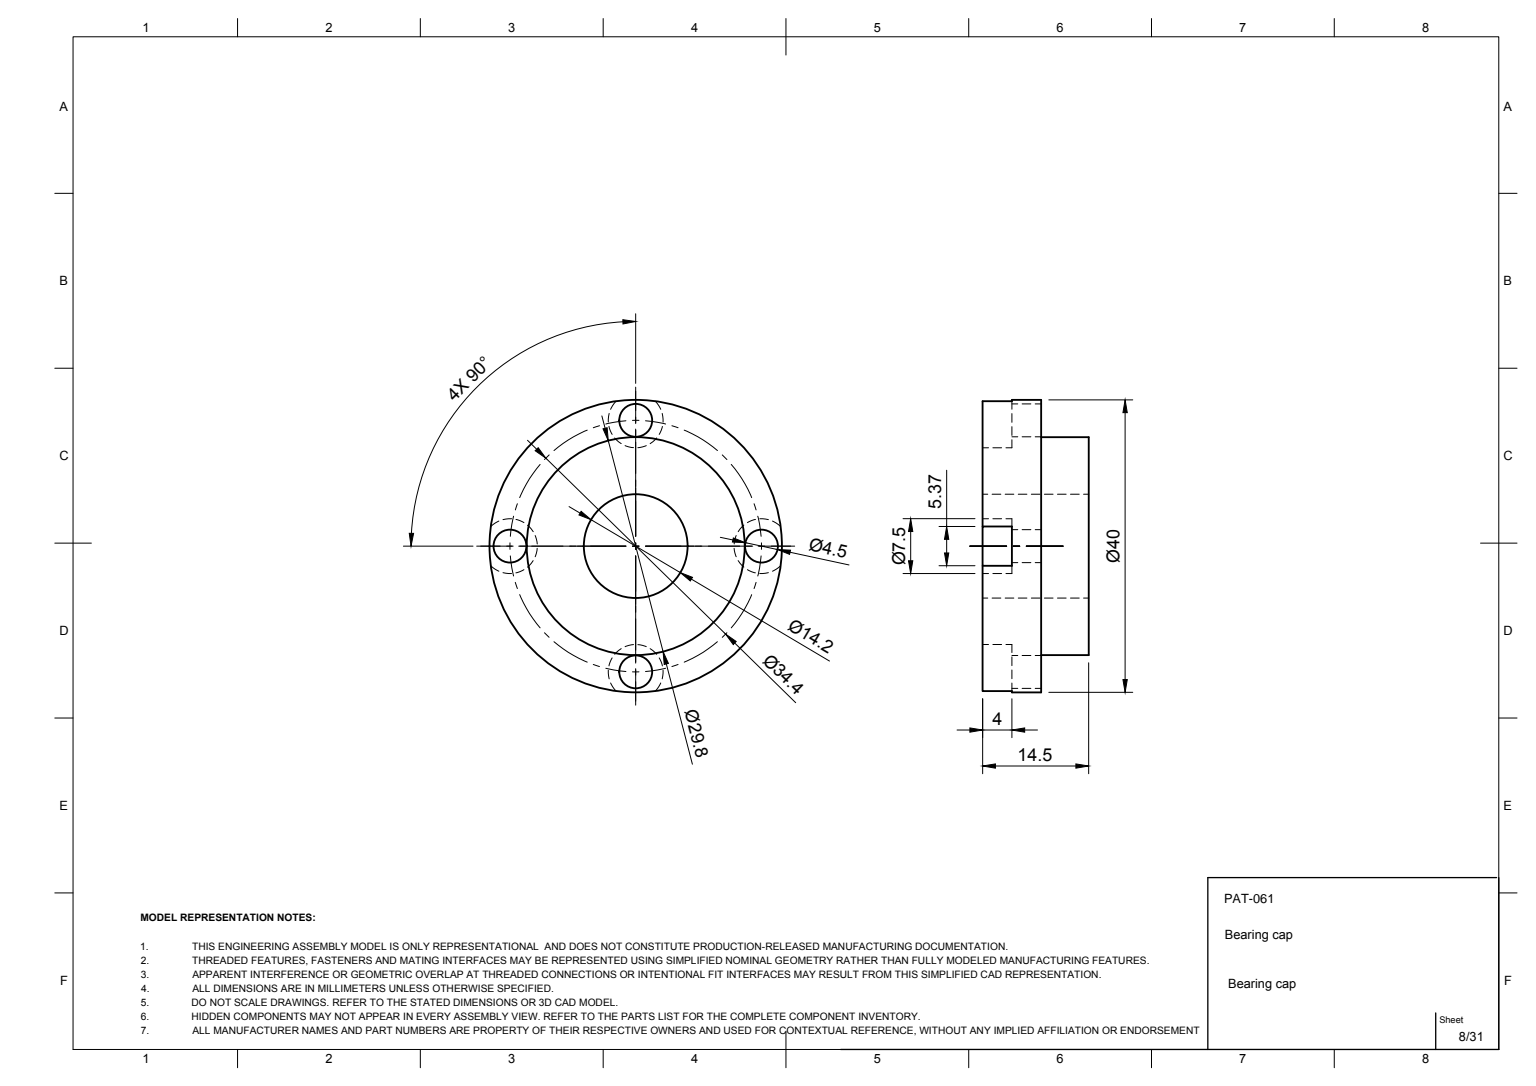
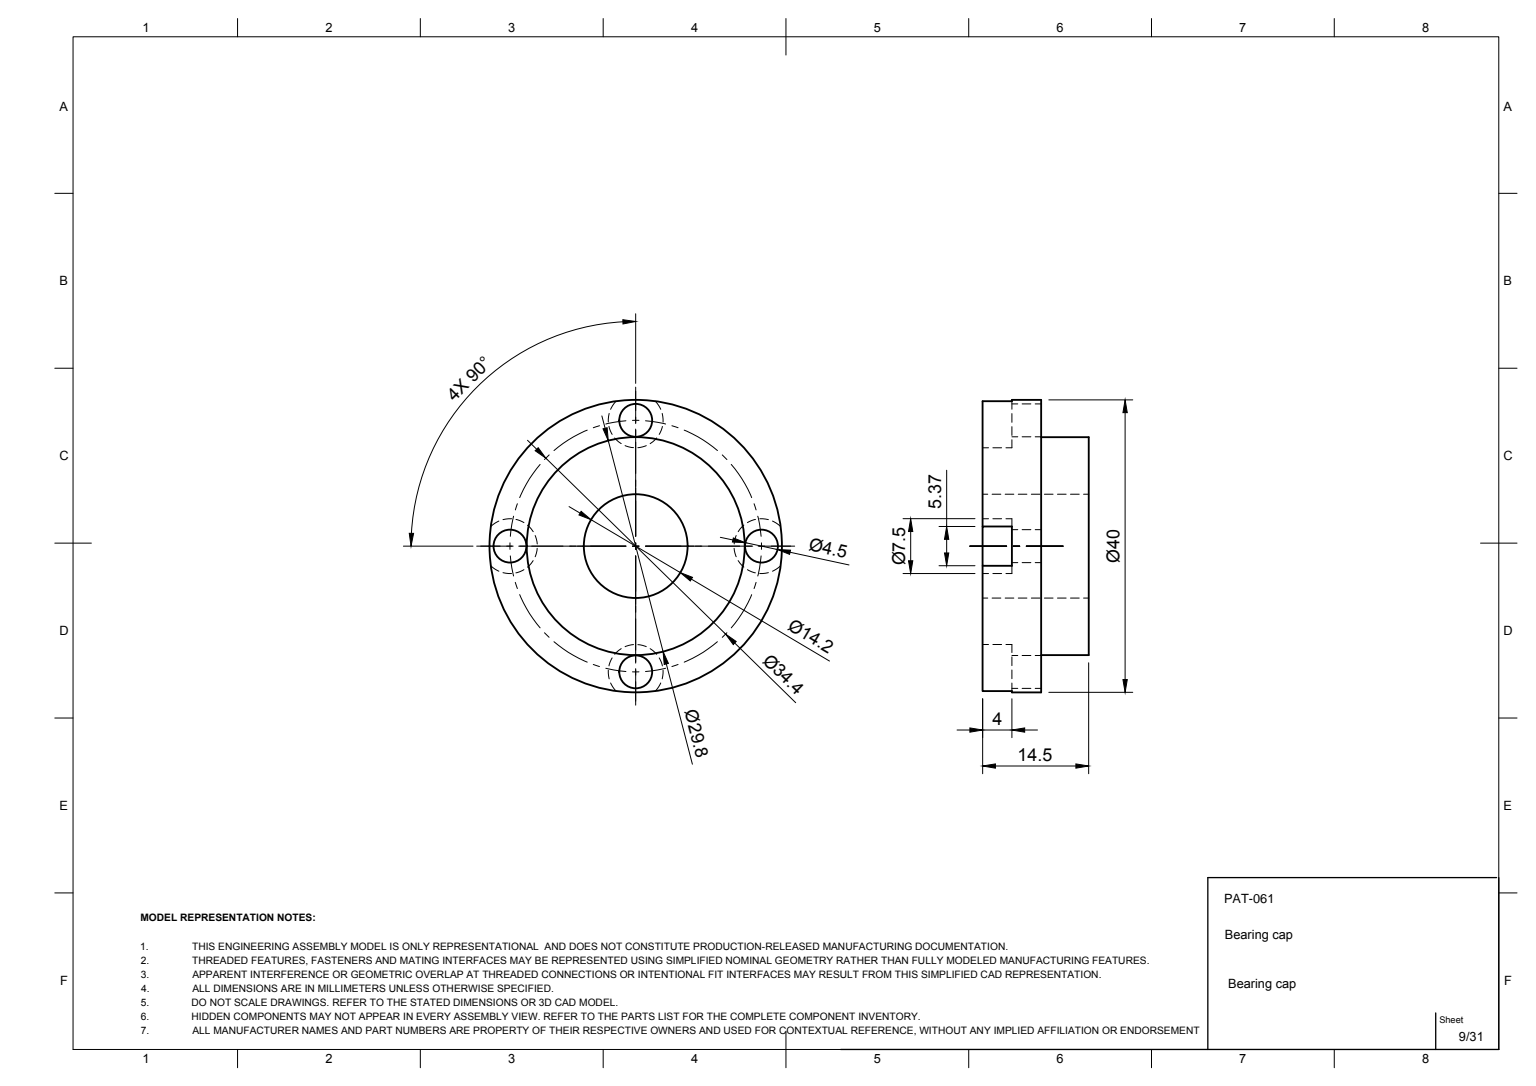
ISO-10303-21;
HEADER;
/* Generated by software containing ST-Developer
 * from STEP Tools, Inc. (www.steptools.com) 
 */

FILE_DESCRIPTION(
/* description */ ('Compact intermittent indexer'),
/* implementation_level */ '2;1');

FILE_NAME(
/* name */ 'Bearing cap.step',
/* time_stamp */ '2026-10-29T16:32:17-07:00',
/* author */ (''),
/* organization */ (''),
/* preprocessor_version */ 'ST-DEVELOPER v20.2',
/* originating_system */ 'Autodesk Translation Framework v15.17.0.0',
/* authorisation */ '');

FILE_SCHEMA (('AUTOMOTIVE_DESIGN { 1 0 10303 214 3 1 1 }'));
ENDSEC;

DATA;
#10=MECHANICAL_DESIGN_GEOMETRIC_PRESENTATION_REPRESENTATION('',(#260),#10837);
#212=SHAPE_REPRESENTATION_RELATIONSHIP('SRR','None',#10946,#236);
#236=ADVANCED_BREP_SHAPE_REPRESENTATION('',(#292),#10813);
#260=STYLED_ITEM('',(#11166),#292);
#292=MANIFOLD_SOLID_BREP('Body1',#5632);
#400=FACE_BOUND('',#1102,.T.);
#401=FACE_BOUND('',#1104,.T.);
#402=FACE_BOUND('',#1107,.T.);
#403=FACE_BOUND('',#1110,.T.);
#404=FACE_BOUND('',#1113,.T.);
#405=FACE_BOUND('',#1120,.T.);
#406=FACE_BOUND('',#1124,.T.);
#407=FACE_BOUND('',#1125,.T.);
#408=FACE_BOUND('',#1126,.T.);
#409=FACE_BOUND('',#1127,.T.);
#410=FACE_BOUND('',#1128,.T.);
#514=PLANE('',#6068);
#515=PLANE('',#6072);
#516=PLANE('',#6078);
#517=PLANE('',#6084);
#518=PLANE('',#6090);
#519=PLANE('',#6107);
#520=PLANE('',#6112);
#725=FACE_OUTER_BOUND('',#1100,.T.);
#726=FACE_OUTER_BOUND('',#1101,.T.);
#727=FACE_OUTER_BOUND('',#1103,.T.);
#728=FACE_OUTER_BOUND('',#1105,.T.);
#729=FACE_OUTER_BOUND('',#1106,.T.);
#730=FACE_OUTER_BOUND('',#1108,.T.);
#731=FACE_OUTER_BOUND('',#1109,.T.);
#732=FACE_OUTER_BOUND('',#1111,.T.);
#733=FACE_OUTER_BOUND('',#1112,.T.);
#734=FACE_OUTER_BOUND('',#1114,.T.);
#735=FACE_OUTER_BOUND('',#1115,.T.);
#736=FACE_OUTER_BOUND('',#1116,.T.);
#737=FACE_OUTER_BOUND('',#1117,.T.);
#738=FACE_OUTER_BOUND('',#1118,.T.);
#739=FACE_OUTER_BOUND('',#1119,.T.);
#740=FACE_OUTER_BOUND('',#1121,.T.);
#741=FACE_OUTER_BOUND('',#1122,.T.);
#742=FACE_OUTER_BOUND('',#1123,.T.);
#1100=EDGE_LOOP('',(#3984,#3985,#3986,#3987));
#1101=EDGE_LOOP('',(#3988,#3989,#3990));
#1102=EDGE_LOOP('',(#3991));
#1103=EDGE_LOOP('',(#3992,#3993));
#1104=EDGE_LOOP('',(#3994));
#1105=EDGE_LOOP('',(#3995,#3996,#3997,#3998));
#1106=EDGE_LOOP('',(#3999,#4000));
#1107=EDGE_LOOP('',(#4001));
#1108=EDGE_LOOP('',(#4002,#4003,#4004,#4005));
#1109=EDGE_LOOP('',(#4006,#4007));
#1110=EDGE_LOOP('',(#4008));
#1111=EDGE_LOOP('',(#4009,#4010,#4011,#4012));
#1112=EDGE_LOOP('',(#4013,#4014,#4015,#4016,#4017,#4018,#4019,#4020));
#1113=EDGE_LOOP('',(#4021));
#1114=EDGE_LOOP('',(#4022,#4023,#4024,#4025));
#1115=EDGE_LOOP('',(#4026,#4027,#4028,#4029));
#1116=EDGE_LOOP('',(#4030,#4031,#4032,#4033));
#1117=EDGE_LOOP('',(#4034,#4035,#4036,#4037));
#1118=EDGE_LOOP('',(#4038,#4039,#4040,#4041));
#1119=EDGE_LOOP('',(#4042));
#1120=EDGE_LOOP('',(#4043));
#1121=EDGE_LOOP('',(#4044,#4045,#4046,#4047));
#1122=EDGE_LOOP('',(#4048,#4049,#4050,#4051,#4052,#4053,#4054,#4055,#4056,
#4057,#4058,#4059,#4060,#4061,#4062,#4063,#4064,#4065,#4066,#4067));
#1123=EDGE_LOOP('',(#4068));
#1124=EDGE_LOOP('',(#4069));
#1125=EDGE_LOOP('',(#4070));
#1126=EDGE_LOOP('',(#4071));
#1127=EDGE_LOOP('',(#4072));
#1128=EDGE_LOOP('',(#4073));
#1510=LINE('',#8878,#1868);
#1511=LINE('',#8882,#1869);
#1512=LINE('',#8899,#1870);
#1513=LINE('',#8902,#1871);
#1514=LINE('',#8912,#1872);
#1515=LINE('',#8915,#1873);
#1516=LINE('',#8925,#1874);
#1517=LINE('',#8928,#1875);
#1518=LINE('',#8939,#1876);
#1519=LINE('',#8943,#1877);
#1520=LINE('',#8947,#1878);
#1521=LINE('',#8951,#1879);
#1522=LINE('',#8956,#1880);
#1523=LINE('',#8962,#1881);
#1524=LINE('',#8965,#1882);
#1868=VECTOR('',#7020,1.);
#1869=VECTOR('',#7023,1.);
#1870=VECTOR('',#7044,1.);
#1871=VECTOR('',#7047,1.);
#1872=VECTOR('',#7058,1.);
#1873=VECTOR('',#7061,1.);
#1874=VECTOR('',#7072,1.);
#1875=VECTOR('',#7075,1.);
#1876=VECTOR('',#7092,0.225);
#1877=VECTOR('',#7097,0.225);
#1878=VECTOR('',#7102,0.225);
#1879=VECTOR('',#7107,0.225);
#1880=VECTOR('',#7112,1.49);
#1881=VECTOR('',#7121,0.71);
#1882=VECTOR('',#7124,2.);
#2206=CIRCLE('',#6066,0.375);
#2207=CIRCLE('',#6067,0.375);
#2208=CIRCLE('',#6069,2.);
#2209=CIRCLE('',#6070,2.);
#2210=CIRCLE('',#6071,0.225);
#2211=CIRCLE('',#6073,2.);
#2212=CIRCLE('',#6074,0.375);
#2213=CIRCLE('',#6075,0.225);
#2214=CIRCLE('',#6077,0.375);
#2215=CIRCLE('',#6079,2.);
#2216=CIRCLE('',#6080,0.375);
#2217=CIRCLE('',#6081,0.225);
#2218=CIRCLE('',#6083,0.375);
#2219=CIRCLE('',#6085,2.);
#2220=CIRCLE('',#6086,0.375);
#2221=CIRCLE('',#6087,0.225);
#2222=CIRCLE('',#6089,0.375);
#2223=CIRCLE('',#6091,2.);
#2224=CIRCLE('',#6092,2.);
#2225=CIRCLE('',#6093,2.);
#2226=CIRCLE('',#6094,2.);
#2227=CIRCLE('',#6095,0.71);
#2228=CIRCLE('',#6097,0.225);
#2229=CIRCLE('',#6099,0.225);
#2230=CIRCLE('',#6101,0.225);
#2231=CIRCLE('',#6103,0.225);
#2232=CIRCLE('',#6105,1.49);
#2233=CIRCLE('',#6106,1.49);
#2234=CIRCLE('',#6108,0.71);
#2235=CIRCLE('',#6111,2.);
#2574=VERTEX_POINT('',#8876);
#2575=VERTEX_POINT('',#8877);
#2576=VERTEX_POINT('',#8879);
#2577=VERTEX_POINT('',#8881);
#2578=VERTEX_POINT('',#8885);
#2579=VERTEX_POINT('',#8888);
#2580=VERTEX_POINT('',#8891);
#2581=VERTEX_POINT('',#8892);
#2582=VERTEX_POINT('',#8895);
#2583=VERTEX_POINT('',#8898);
#2584=VERTEX_POINT('',#8900);
#2585=VERTEX_POINT('',#8904);
#2586=VERTEX_POINT('',#8905);
#2587=VERTEX_POINT('',#8908);
#2588=VERTEX_POINT('',#8911);
#2589=VERTEX_POINT('',#8913);
#2590=VERTEX_POINT('',#8917);
#2591=VERTEX_POINT('',#8918);
#2592=VERTEX_POINT('',#8921);
#2593=VERTEX_POINT('',#8924);
#2594=VERTEX_POINT('',#8926);
#2595=VERTEX_POINT('',#8934);
#2596=VERTEX_POINT('',#8937);
#2597=VERTEX_POINT('',#8941);
#2598=VERTEX_POINT('',#8945);
#2599=VERTEX_POINT('',#8949);
#2600=VERTEX_POINT('',#8953);
#2601=VERTEX_POINT('',#8955);
#2602=VERTEX_POINT('',#8959);
#2603=VERTEX_POINT('',#8964);
#3114=EDGE_CURVE('',#2574,#2575,#1510,.T.);
#3115=EDGE_CURVE('',#2576,#2574,#2206,.T.);
#3116=EDGE_CURVE('',#2577,#2576,#1511,.T.);
#3117=EDGE_CURVE('',#2575,#2577,#2207,.T.);
#3118=EDGE_CURVE('',#2576,#2578,#2208,.T.);
#3119=EDGE_CURVE('',#2578,#2574,#2209,.T.);
#3120=EDGE_CURVE('',#2579,#2579,#2210,.T.);
#3121=EDGE_CURVE('',#2580,#2581,#2211,.T.);
#3122=EDGE_CURVE('',#2580,#2581,#2212,.T.);
#3123=EDGE_CURVE('',#2582,#2582,#2213,.T.);
#3124=EDGE_CURVE('',#2583,#2580,#1512,.T.);
#3125=EDGE_CURVE('',#2584,#2583,#2214,.T.);
#3126=EDGE_CURVE('',#2581,#2584,#1513,.T.);
#3127=EDGE_CURVE('',#2585,#2586,#2215,.T.);
#3128=EDGE_CURVE('',#2585,#2586,#2216,.T.);
#3129=EDGE_CURVE('',#2587,#2587,#2217,.T.);
#3130=EDGE_CURVE('',#2588,#2585,#1514,.T.);
#3131=EDGE_CURVE('',#2589,#2588,#2218,.T.);
#3132=EDGE_CURVE('',#2586,#2589,#1515,.T.);
#3133=EDGE_CURVE('',#2590,#2591,#2219,.T.);
#3134=EDGE_CURVE('',#2590,#2591,#2220,.T.);
#3135=EDGE_CURVE('',#2592,#2592,#2221,.T.);
#3136=EDGE_CURVE('',#2593,#2590,#1516,.T.);
#3137=EDGE_CURVE('',#2594,#2593,#2222,.T.);
#3138=EDGE_CURVE('',#2591,#2594,#1517,.T.);
#3139=EDGE_CURVE('',#2577,#2594,#2223,.T.);
#3140=EDGE_CURVE('',#2593,#2589,#2224,.T.);
#3141=EDGE_CURVE('',#2588,#2584,#2225,.T.);
#3142=EDGE_CURVE('',#2583,#2575,#2226,.T.);
#3143=EDGE_CURVE('',#2595,#2595,#2227,.T.);
#3144=EDGE_CURVE('',#2596,#2596,#2228,.T.);
#3145=EDGE_CURVE('',#2596,#2579,#1518,.T.);
#3146=EDGE_CURVE('',#2597,#2597,#2229,.T.);
#3147=EDGE_CURVE('',#2597,#2582,#1519,.T.);
#3148=EDGE_CURVE('',#2598,#2598,#2230,.T.);
#3149=EDGE_CURVE('',#2598,#2587,#1520,.T.);
#3150=EDGE_CURVE('',#2599,#2599,#2231,.T.);
#3151=EDGE_CURVE('',#2599,#2592,#1521,.T.);
#3152=EDGE_CURVE('',#2600,#2600,#2232,.T.);
#3153=EDGE_CURVE('',#2600,#2601,#1522,.T.);
#3154=EDGE_CURVE('',#2601,#2601,#2233,.T.);
#3155=EDGE_CURVE('',#2602,#2602,#2234,.T.);
#3156=EDGE_CURVE('',#2595,#2602,#1523,.T.);
#3157=EDGE_CURVE('',#2578,#2603,#1524,.T.);
#3158=EDGE_CURVE('',#2603,#2603,#2235,.T.);
#3984=ORIENTED_EDGE('',*,*,#3114,.F.);
#3985=ORIENTED_EDGE('',*,*,#3115,.F.);
#3986=ORIENTED_EDGE('',*,*,#3116,.F.);
#3987=ORIENTED_EDGE('',*,*,#3117,.F.);
#3988=ORIENTED_EDGE('',*,*,#3118,.F.);
#3989=ORIENTED_EDGE('',*,*,#3115,.T.);
#3990=ORIENTED_EDGE('',*,*,#3119,.F.);
#3991=ORIENTED_EDGE('',*,*,#3120,.F.);
#3992=ORIENTED_EDGE('',*,*,#3121,.F.);
#3993=ORIENTED_EDGE('',*,*,#3122,.T.);
#3994=ORIENTED_EDGE('',*,*,#3123,.F.);
#3995=ORIENTED_EDGE('',*,*,#3124,.F.);
#3996=ORIENTED_EDGE('',*,*,#3125,.F.);
#3997=ORIENTED_EDGE('',*,*,#3126,.F.);
#3998=ORIENTED_EDGE('',*,*,#3122,.F.);
#3999=ORIENTED_EDGE('',*,*,#3127,.F.);
#4000=ORIENTED_EDGE('',*,*,#3128,.T.);
#4001=ORIENTED_EDGE('',*,*,#3129,.F.);
#4002=ORIENTED_EDGE('',*,*,#3130,.F.);
#4003=ORIENTED_EDGE('',*,*,#3131,.F.);
#4004=ORIENTED_EDGE('',*,*,#3132,.F.);
#4005=ORIENTED_EDGE('',*,*,#3128,.F.);
#4006=ORIENTED_EDGE('',*,*,#3133,.F.);
#4007=ORIENTED_EDGE('',*,*,#3134,.T.);
#4008=ORIENTED_EDGE('',*,*,#3135,.F.);
#4009=ORIENTED_EDGE('',*,*,#3136,.F.);
#4010=ORIENTED_EDGE('',*,*,#3137,.F.);
#4011=ORIENTED_EDGE('',*,*,#3138,.F.);
#4012=ORIENTED_EDGE('',*,*,#3134,.F.);
#4013=ORIENTED_EDGE('',*,*,#3117,.T.);
#4014=ORIENTED_EDGE('',*,*,#3139,.T.);
#4015=ORIENTED_EDGE('',*,*,#3137,.T.);
#4016=ORIENTED_EDGE('',*,*,#3140,.T.);
#4017=ORIENTED_EDGE('',*,*,#3131,.T.);
#4018=ORIENTED_EDGE('',*,*,#3141,.T.);
#4019=ORIENTED_EDGE('',*,*,#3125,.T.);
#4020=ORIENTED_EDGE('',*,*,#3142,.T.);
#4021=ORIENTED_EDGE('',*,*,#3143,.T.);
#4022=ORIENTED_EDGE('',*,*,#3144,.F.);
#4023=ORIENTED_EDGE('',*,*,#3145,.T.);
#4024=ORIENTED_EDGE('',*,*,#3120,.T.);
#4025=ORIENTED_EDGE('',*,*,#3145,.F.);
#4026=ORIENTED_EDGE('',*,*,#3146,.F.);
#4027=ORIENTED_EDGE('',*,*,#3147,.T.);
#4028=ORIENTED_EDGE('',*,*,#3123,.T.);
#4029=ORIENTED_EDGE('',*,*,#3147,.F.);
#4030=ORIENTED_EDGE('',*,*,#3148,.F.);
#4031=ORIENTED_EDGE('',*,*,#3149,.T.);
#4032=ORIENTED_EDGE('',*,*,#3129,.T.);
#4033=ORIENTED_EDGE('',*,*,#3149,.F.);
#4034=ORIENTED_EDGE('',*,*,#3150,.F.);
#4035=ORIENTED_EDGE('',*,*,#3151,.T.);
#4036=ORIENTED_EDGE('',*,*,#3135,.T.);
#4037=ORIENTED_EDGE('',*,*,#3151,.F.);
#4038=ORIENTED_EDGE('',*,*,#3152,.F.);
#4039=ORIENTED_EDGE('',*,*,#3153,.T.);
#4040=ORIENTED_EDGE('',*,*,#3154,.T.);
#4041=ORIENTED_EDGE('',*,*,#3153,.F.);
#4042=ORIENTED_EDGE('',*,*,#3154,.F.);
#4043=ORIENTED_EDGE('',*,*,#3155,.F.);
#4044=ORIENTED_EDGE('',*,*,#3143,.F.);
#4045=ORIENTED_EDGE('',*,*,#3156,.T.);
#4046=ORIENTED_EDGE('',*,*,#3155,.T.);
#4047=ORIENTED_EDGE('',*,*,#3156,.F.);
#4048=ORIENTED_EDGE('',*,*,#3114,.T.);
#4049=ORIENTED_EDGE('',*,*,#3142,.F.);
#4050=ORIENTED_EDGE('',*,*,#3124,.T.);
#4051=ORIENTED_EDGE('',*,*,#3121,.T.);
#4052=ORIENTED_EDGE('',*,*,#3126,.T.);
#4053=ORIENTED_EDGE('',*,*,#3141,.F.);
#4054=ORIENTED_EDGE('',*,*,#3130,.T.);
#4055=ORIENTED_EDGE('',*,*,#3127,.T.);
#4056=ORIENTED_EDGE('',*,*,#3132,.T.);
#4057=ORIENTED_EDGE('',*,*,#3140,.F.);
#4058=ORIENTED_EDGE('',*,*,#3136,.T.);
#4059=ORIENTED_EDGE('',*,*,#3133,.T.);
#4060=ORIENTED_EDGE('',*,*,#3138,.T.);
#4061=ORIENTED_EDGE('',*,*,#3139,.F.);
#4062=ORIENTED_EDGE('',*,*,#3116,.T.);
#4063=ORIENTED_EDGE('',*,*,#3118,.T.);
#4064=ORIENTED_EDGE('',*,*,#3157,.T.);
#4065=ORIENTED_EDGE('',*,*,#3158,.T.);
#4066=ORIENTED_EDGE('',*,*,#3157,.F.);
#4067=ORIENTED_EDGE('',*,*,#3119,.T.);
#4068=ORIENTED_EDGE('',*,*,#3158,.F.);
#4069=ORIENTED_EDGE('',*,*,#3152,.T.);
#4070=ORIENTED_EDGE('',*,*,#3150,.T.);
#4071=ORIENTED_EDGE('',*,*,#3148,.T.);
#4072=ORIENTED_EDGE('',*,*,#3146,.T.);
#4073=ORIENTED_EDGE('',*,*,#3144,.T.);
#5202=CYLINDRICAL_SURFACE('',#6065,0.375);
#5203=CYLINDRICAL_SURFACE('',#6076,0.375);
#5204=CYLINDRICAL_SURFACE('',#6082,0.375);
#5205=CYLINDRICAL_SURFACE('',#6088,0.375);
#5206=CYLINDRICAL_SURFACE('',#6096,0.225);
#5207=CYLINDRICAL_SURFACE('',#6098,0.225);
#5208=CYLINDRICAL_SURFACE('',#6100,0.225);
#5209=CYLINDRICAL_SURFACE('',#6102,0.225);
#5210=CYLINDRICAL_SURFACE('',#6104,1.49);
#5211=CYLINDRICAL_SURFACE('',#6109,0.71);
#5212=CYLINDRICAL_SURFACE('',#6110,2.);
#5368=ADVANCED_FACE('',(#725),#5202,.F.);
#5369=ADVANCED_FACE('',(#726,#400),#514,.T.);
#5370=ADVANCED_FACE('',(#727,#401),#515,.T.);
#5371=ADVANCED_FACE('',(#728),#5203,.F.);
#5372=ADVANCED_FACE('',(#729,#402),#516,.T.);
#5373=ADVANCED_FACE('',(#730),#5204,.F.);
#5374=ADVANCED_FACE('',(#731,#403),#517,.T.);
#5375=ADVANCED_FACE('',(#732),#5205,.F.);
#5376=ADVANCED_FACE('',(#733,#404),#518,.T.);
#5377=ADVANCED_FACE('',(#734),#5206,.F.);
#5378=ADVANCED_FACE('',(#735),#5207,.F.);
#5379=ADVANCED_FACE('',(#736),#5208,.F.);
#5380=ADVANCED_FACE('',(#737),#5209,.F.);
#5381=ADVANCED_FACE('',(#738),#5210,.T.);
#5382=ADVANCED_FACE('',(#739,#405),#519,.F.);
#5383=ADVANCED_FACE('',(#740),#5211,.F.);
#5384=ADVANCED_FACE('',(#741),#5212,.T.);
#5385=ADVANCED_FACE('',(#742,#406,#407,#408,#409,#410),#520,.F.);
#5632=CLOSED_SHELL('',(#5368,#5369,#5370,#5371,#5372,#5373,#5374,#5375,
#5376,#5377,#5378,#5379,#5380,#5381,#5382,#5383,#5384,#5385));
#6064=AXIS2_PLACEMENT_3D('',#8874,#7016,#7017);
#6065=AXIS2_PLACEMENT_3D('',#8875,#7018,#7019);
#6066=AXIS2_PLACEMENT_3D('',#8880,#7021,#7022);
#6067=AXIS2_PLACEMENT_3D('',#8883,#7024,#7025);
#6068=AXIS2_PLACEMENT_3D('',#8884,#7026,#7027);
#6069=AXIS2_PLACEMENT_3D('',#8886,#7028,#7029);
#6070=AXIS2_PLACEMENT_3D('',#8887,#7030,#7031);
#6071=AXIS2_PLACEMENT_3D('',#8889,#7032,#7033);
#6072=AXIS2_PLACEMENT_3D('',#8890,#7034,#7035);
#6073=AXIS2_PLACEMENT_3D('',#8893,#7036,#7037);
#6074=AXIS2_PLACEMENT_3D('',#8894,#7038,#7039);
#6075=AXIS2_PLACEMENT_3D('',#8896,#7040,#7041);
#6076=AXIS2_PLACEMENT_3D('',#8897,#7042,#7043);
#6077=AXIS2_PLACEMENT_3D('',#8901,#7045,#7046);
#6078=AXIS2_PLACEMENT_3D('',#8903,#7048,#7049);
#6079=AXIS2_PLACEMENT_3D('',#8906,#7050,#7051);
#6080=AXIS2_PLACEMENT_3D('',#8907,#7052,#7053);
#6081=AXIS2_PLACEMENT_3D('',#8909,#7054,#7055);
#6082=AXIS2_PLACEMENT_3D('',#8910,#7056,#7057);
#6083=AXIS2_PLACEMENT_3D('',#8914,#7059,#7060);
#6084=AXIS2_PLACEMENT_3D('',#8916,#7062,#7063);
#6085=AXIS2_PLACEMENT_3D('',#8919,#7064,#7065);
#6086=AXIS2_PLACEMENT_3D('',#8920,#7066,#7067);
#6087=AXIS2_PLACEMENT_3D('',#8922,#7068,#7069);
#6088=AXIS2_PLACEMENT_3D('',#8923,#7070,#7071);
#6089=AXIS2_PLACEMENT_3D('',#8927,#7073,#7074);
#6090=AXIS2_PLACEMENT_3D('',#8929,#7076,#7077);
#6091=AXIS2_PLACEMENT_3D('',#8930,#7078,#7079);
#6092=AXIS2_PLACEMENT_3D('',#8931,#7080,#7081);
#6093=AXIS2_PLACEMENT_3D('',#8932,#7082,#7083);
#6094=AXIS2_PLACEMENT_3D('',#8933,#7084,#7085);
#6095=AXIS2_PLACEMENT_3D('',#8935,#7086,#7087);
#6096=AXIS2_PLACEMENT_3D('',#8936,#7088,#7089);
#6097=AXIS2_PLACEMENT_3D('',#8938,#7090,#7091);
#6098=AXIS2_PLACEMENT_3D('',#8940,#7093,#7094);
#6099=AXIS2_PLACEMENT_3D('',#8942,#7095,#7096);
#6100=AXIS2_PLACEMENT_3D('',#8944,#7098,#7099);
#6101=AXIS2_PLACEMENT_3D('',#8946,#7100,#7101);
#6102=AXIS2_PLACEMENT_3D('',#8948,#7103,#7104);
#6103=AXIS2_PLACEMENT_3D('',#8950,#7105,#7106);
#6104=AXIS2_PLACEMENT_3D('',#8952,#7108,#7109);
#6105=AXIS2_PLACEMENT_3D('',#8954,#7110,#7111);
#6106=AXIS2_PLACEMENT_3D('',#8957,#7113,#7114);
#6107=AXIS2_PLACEMENT_3D('',#8958,#7115,#7116);
#6108=AXIS2_PLACEMENT_3D('',#8960,#7117,#7118);
#6109=AXIS2_PLACEMENT_3D('',#8961,#7119,#7120);
#6110=AXIS2_PLACEMENT_3D('',#8963,#7122,#7123);
#6111=AXIS2_PLACEMENT_3D('',#8966,#7125,#7126);
#6112=AXIS2_PLACEMENT_3D('',#8967,#7127,#7128);
#7016=DIRECTION('axis',(0.,0.,1.));
#7017=DIRECTION('refdir',(1.,0.,0.));
#7018=DIRECTION('center_axis',(0.,0.,1.));
#7019=DIRECTION('ref_axis',(1.,0.,0.));
#7020=DIRECTION('',(0.,0.,1.));
#7021=DIRECTION('center_axis',(0.,0.,1.));
#7022=DIRECTION('ref_axis',(1.,0.,0.));
#7023=DIRECTION('',(0.,0.,-1.));
#7024=DIRECTION('center_axis',(0.,0.,-1.));
#7025=DIRECTION('ref_axis',(1.,0.,0.));
#7026=DIRECTION('center_axis',(0.,0.,1.));
#7027=DIRECTION('ref_axis',(1.,0.,0.));
#7028=DIRECTION('center_axis',(0.,0.,-1.));
#7029=DIRECTION('ref_axis',(1.,0.,0.));
#7030=DIRECTION('center_axis',(0.,0.,-1.));
#7031=DIRECTION('ref_axis',(1.,0.,0.));
#7032=DIRECTION('center_axis',(0.,0.,1.));
#7033=DIRECTION('ref_axis',(1.,0.,0.));
#7034=DIRECTION('center_axis',(0.,0.,1.));
#7035=DIRECTION('ref_axis',(1.,0.,0.));
#7036=DIRECTION('center_axis',(0.,0.,-1.));
#7037=DIRECTION('ref_axis',(1.,0.,0.));
#7038=DIRECTION('center_axis',(0.,0.,1.));
#7039=DIRECTION('ref_axis',(1.,0.,0.));
#7040=DIRECTION('center_axis',(0.,0.,1.));
#7041=DIRECTION('ref_axis',(1.,0.,0.));
#7042=DIRECTION('center_axis',(0.,0.,1.));
#7043=DIRECTION('ref_axis',(-1.83697019872103E-16,-1.,0.));
#7044=DIRECTION('',(0.,0.,-1.));
#7045=DIRECTION('center_axis',(0.,0.,-1.));
#7046=DIRECTION('ref_axis',(1.,0.,0.));
#7047=DIRECTION('',(0.,0.,1.));
#7048=DIRECTION('center_axis',(0.,0.,1.));
#7049=DIRECTION('ref_axis',(1.,0.,0.));
#7050=DIRECTION('center_axis',(0.,0.,-1.));
#7051=DIRECTION('ref_axis',(1.,0.,0.));
#7052=DIRECTION('center_axis',(0.,0.,1.));
#7053=DIRECTION('ref_axis',(1.,0.,0.));
#7054=DIRECTION('center_axis',(0.,0.,1.));
#7055=DIRECTION('ref_axis',(1.,0.,0.));
#7056=DIRECTION('center_axis',(0.,0.,1.));
#7057=DIRECTION('ref_axis',(-1.,1.22464679914735E-16,0.));
#7058=DIRECTION('',(0.,0.,-1.));
#7059=DIRECTION('center_axis',(0.,0.,-1.));
#7060=DIRECTION('ref_axis',(1.,0.,0.));
#7061=DIRECTION('',(0.,0.,1.));
#7062=DIRECTION('center_axis',(0.,0.,1.));
#7063=DIRECTION('ref_axis',(1.,0.,0.));
#7064=DIRECTION('center_axis',(0.,0.,-1.));
#7065=DIRECTION('ref_axis',(1.,0.,0.));
#7066=DIRECTION('center_axis',(0.,0.,1.));
#7067=DIRECTION('ref_axis',(1.,0.,0.));
#7068=DIRECTION('center_axis',(0.,0.,1.));
#7069=DIRECTION('ref_axis',(1.,0.,0.));
#7070=DIRECTION('center_axis',(0.,0.,1.));
#7071=DIRECTION('ref_axis',(6.12323399573677E-17,1.,0.));
#7072=DIRECTION('',(0.,0.,-1.));
#7073=DIRECTION('center_axis',(0.,0.,-1.));
#7074=DIRECTION('ref_axis',(1.,0.,0.));
#7075=DIRECTION('',(0.,0.,1.));
#7076=DIRECTION('center_axis',(0.,0.,1.));
#7077=DIRECTION('ref_axis',(1.,0.,0.));
#7078=DIRECTION('center_axis',(0.,0.,1.));
#7079=DIRECTION('ref_axis',(1.,0.,0.));
#7080=DIRECTION('center_axis',(0.,0.,1.));
#7081=DIRECTION('ref_axis',(1.,0.,0.));
#7082=DIRECTION('center_axis',(0.,0.,1.));
#7083=DIRECTION('ref_axis',(1.,0.,0.));
#7084=DIRECTION('center_axis',(0.,0.,1.));
#7085=DIRECTION('ref_axis',(1.,0.,0.));
#7086=DIRECTION('center_axis',(0.,0.,-1.));
#7087=DIRECTION('ref_axis',(1.,0.,0.));
#7088=DIRECTION('center_axis',(0.,0.,1.));
#7089=DIRECTION('ref_axis',(1.,0.,0.));
#7090=DIRECTION('center_axis',(0.,0.,1.));
#7091=DIRECTION('ref_axis',(1.,0.,0.));
#7092=DIRECTION('',(0.,0.,1.));
#7093=DIRECTION('center_axis',(0.,0.,1.));
#7094=DIRECTION('ref_axis',(1.,0.,0.));
#7095=DIRECTION('center_axis',(0.,0.,1.));
#7096=DIRECTION('ref_axis',(1.,0.,0.));
#7097=DIRECTION('',(0.,0.,1.));
#7098=DIRECTION('center_axis',(0.,0.,1.));
#7099=DIRECTION('ref_axis',(1.,0.,0.));
#7100=DIRECTION('center_axis',(0.,0.,1.));
#7101=DIRECTION('ref_axis',(1.,0.,0.));
#7102=DIRECTION('',(0.,0.,1.));
#7103=DIRECTION('center_axis',(0.,0.,1.));
#7104=DIRECTION('ref_axis',(1.,0.,0.));
#7105=DIRECTION('center_axis',(0.,0.,1.));
#7106=DIRECTION('ref_axis',(1.,0.,0.));
#7107=DIRECTION('',(0.,0.,1.));
#7108=DIRECTION('center_axis',(0.,0.,1.));
#7109=DIRECTION('ref_axis',(1.,0.,0.));
#7110=DIRECTION('center_axis',(0.,0.,1.));
#7111=DIRECTION('ref_axis',(1.,0.,0.));
#7112=DIRECTION('',(0.,0.,-1.));
#7113=DIRECTION('center_axis',(0.,0.,1.));
#7114=DIRECTION('ref_axis',(1.,0.,0.));
#7115=DIRECTION('center_axis',(0.,0.,1.));
#7116=DIRECTION('ref_axis',(1.,0.,0.));
#7117=DIRECTION('center_axis',(0.,0.,-1.));
#7118=DIRECTION('ref_axis',(1.,0.,0.));
#7119=DIRECTION('center_axis',(0.,0.,1.));
#7120=DIRECTION('ref_axis',(1.,0.,0.));
#7121=DIRECTION('',(0.,0.,-1.));
#7122=DIRECTION('center_axis',(0.,0.,1.));
#7123=DIRECTION('ref_axis',(1.,0.,0.));
#7124=DIRECTION('',(0.,0.,-1.));
#7125=DIRECTION('center_axis',(0.,0.,1.));
#7126=DIRECTION('ref_axis',(1.,0.,0.));
#7127=DIRECTION('center_axis',(0.,0.,1.));
#7128=DIRECTION('ref_axis',(1.,0.,0.));
#8874=CARTESIAN_POINT('',(0.,0.,0.));
#8875=CARTESIAN_POINT('Origin',(-1.72,2.10639249453345E-16,4.));
#8876=CARTESIAN_POINT('',(-1.9819113372093,0.268379305165721,4.));
#8877=CARTESIAN_POINT('',(-1.9819113372093,0.26837930516572,4.4));
#8878=CARTESIAN_POINT('',(-1.9819113372093,0.268379305165721,4.));
#8879=CARTESIAN_POINT('',(-1.9819113372093,-0.268379305165721,4.));
#8880=CARTESIAN_POINT('Origin',(-1.72,2.10639249453345E-16,4.));
#8881=CARTESIAN_POINT('',(-1.9819113372093,-0.268379305165719,4.4));
#8882=CARTESIAN_POINT('',(-1.9819113372093,-0.268379305165721,4.));
#8883=CARTESIAN_POINT('Origin',(-1.72,2.10639249453345E-16,4.4));
#8884=CARTESIAN_POINT('Origin',(-1.72,2.22044604925031E-16,4.));
#8885=CARTESIAN_POINT('',(-2.,-2.44929359829471E-16,4.));
#8886=CARTESIAN_POINT('Origin',(0.,0.,4.));
#8887=CARTESIAN_POINT('Origin',(0.,0.,4.));
#8888=CARTESIAN_POINT('',(-1.945,1.83084696472529E-16,4.));
#8889=CARTESIAN_POINT('Origin',(-1.72,2.10639249453345E-16,4.));
#8890=CARTESIAN_POINT('Origin',(1.11022302462516E-16,1.72,4.));
#8891=CARTESIAN_POINT('',(-0.268379305165721,1.9819113372093,4.));
#8892=CARTESIAN_POINT('',(0.268379305165721,1.9819113372093,4.));
#8893=CARTESIAN_POINT('Origin',(0.,0.,4.));
#8894=CARTESIAN_POINT('Origin',(1.05319624726672E-16,1.72,4.));
#8895=CARTESIAN_POINT('',(-0.225,1.72,4.));
#8896=CARTESIAN_POINT('Origin',(1.05319624726672E-16,1.72,4.));
#8897=CARTESIAN_POINT('Origin',(1.05319624726672E-16,1.72,4.));
#8898=CARTESIAN_POINT('',(-0.26837930516572,1.9819113372093,4.4));
#8899=CARTESIAN_POINT('',(-0.268379305165721,1.9819113372093,4.));
#8900=CARTESIAN_POINT('',(0.26837930516572,1.9819113372093,4.4));
#8901=CARTESIAN_POINT('Origin',(1.05319624726672E-16,1.72,4.4));
#8902=CARTESIAN_POINT('',(0.268379305165721,1.9819113372093,4.));
#8903=CARTESIAN_POINT('Origin',(1.72,0.,4.));
#8904=CARTESIAN_POINT('',(1.9819113372093,0.268379305165721,4.));
#8905=CARTESIAN_POINT('',(1.9819113372093,-0.268379305165721,4.));
#8906=CARTESIAN_POINT('Origin',(0.,0.,4.));
#8907=CARTESIAN_POINT('Origin',(1.72,0.,4.));
#8908=CARTESIAN_POINT('',(1.495,-2.75545529808155E-17,4.));
#8909=CARTESIAN_POINT('Origin',(1.72,0.,4.));
#8910=CARTESIAN_POINT('Origin',(1.72,0.,4.));
#8911=CARTESIAN_POINT('',(1.9819113372093,0.26837930516572,4.4));
#8912=CARTESIAN_POINT('',(1.9819113372093,0.268379305165721,4.));
#8913=CARTESIAN_POINT('',(1.9819113372093,-0.26837930516572,4.4));
#8914=CARTESIAN_POINT('Origin',(1.72,0.,4.4));
#8915=CARTESIAN_POINT('',(1.9819113372093,-0.268379305165721,4.));
#8916=CARTESIAN_POINT('Origin',(-3.33066907387547E-16,-1.72,4.));
#8917=CARTESIAN_POINT('',(0.26837930516572,-1.9819113372093,4.));
#8918=CARTESIAN_POINT('',(-0.268379305165721,-1.9819113372093,4.));
#8919=CARTESIAN_POINT('Origin',(0.,0.,4.));
#8920=CARTESIAN_POINT('Origin',(-3.15958874180017E-16,-1.72,4.));
#8921=CARTESIAN_POINT('',(-0.225,-1.72,4.));
#8922=CARTESIAN_POINT('Origin',(-3.15958874180017E-16,-1.72,4.));
#8923=CARTESIAN_POINT('Origin',(-3.15958874180017E-16,-1.72,4.));
#8924=CARTESIAN_POINT('',(0.268379305165719,-1.9819113372093,4.4));
#8925=CARTESIAN_POINT('',(0.26837930516572,-1.9819113372093,4.));
#8926=CARTESIAN_POINT('',(-0.26837930516572,-1.9819113372093,4.4));
#8927=CARTESIAN_POINT('Origin',(-3.15958874180017E-16,-1.72,4.4));
#8928=CARTESIAN_POINT('',(-0.268379305165721,-1.9819113372093,4.));
#8929=CARTESIAN_POINT('Origin',(0.,0.,4.4));
#8930=CARTESIAN_POINT('Origin',(0.,0.,4.4));
#8931=CARTESIAN_POINT('Origin',(0.,0.,4.4));
#8932=CARTESIAN_POINT('Origin',(0.,0.,4.4));
#8933=CARTESIAN_POINT('Origin',(0.,0.,4.4));
#8934=CARTESIAN_POINT('',(-0.71,-8.69499227394621E-17,4.4));
#8935=CARTESIAN_POINT('Origin',(0.,0.,4.4));
#8936=CARTESIAN_POINT('Origin',(-1.72,2.10639249453345E-16,3.5));
#8937=CARTESIAN_POINT('',(-1.945,1.83084696472529E-16,3.6));
#8938=CARTESIAN_POINT('Origin',(-1.72,2.10639249453345E-16,3.6));
#8939=CARTESIAN_POINT('',(-1.945,1.83084696472529E-16,3.5));
#8940=CARTESIAN_POINT('Origin',(1.05319624726672E-16,1.72,3.5));
#8941=CARTESIAN_POINT('',(-0.225,1.72,3.6));
#8942=CARTESIAN_POINT('Origin',(1.05319624726672E-16,1.72,3.6));
#8943=CARTESIAN_POINT('',(-0.225,1.72,3.5));
#8944=CARTESIAN_POINT('Origin',(1.72,0.,3.5));
#8945=CARTESIAN_POINT('',(1.495,-2.75545529808155E-17,3.6));
#8946=CARTESIAN_POINT('Origin',(1.72,0.,3.6));
#8947=CARTESIAN_POINT('',(1.495,-2.75545529808155E-17,3.5));
#8948=CARTESIAN_POINT('Origin',(-3.15958874180017E-16,-1.72,3.5));
#8949=CARTESIAN_POINT('',(-0.225,-1.72,3.6));
#8950=CARTESIAN_POINT('Origin',(-3.15958874180017E-16,-1.72,3.6));
#8951=CARTESIAN_POINT('',(-0.225,-1.72,3.5));
#8952=CARTESIAN_POINT('Origin',(0.,0.,2.95));
#8953=CARTESIAN_POINT('',(-1.49,-1.82472373072956E-16,3.6));
#8954=CARTESIAN_POINT('Origin',(0.,0.,3.6));
#8955=CARTESIAN_POINT('',(-1.49,-1.82472373072956E-16,2.95));
#8956=CARTESIAN_POINT('',(-1.49,-1.82472373072956E-16,2.95));
#8957=CARTESIAN_POINT('Origin',(0.,0.,2.95));
#8958=CARTESIAN_POINT('Origin',(0.,0.,2.95));
#8959=CARTESIAN_POINT('',(-0.71,-8.69499227394621E-17,2.95));
#8960=CARTESIAN_POINT('Origin',(0.,0.,2.95));
#8961=CARTESIAN_POINT('Origin',(0.,0.,3.6));
#8962=CARTESIAN_POINT('',(-0.71,-8.69499227394621E-17,3.6));
#8963=CARTESIAN_POINT('Origin',(0.,0.,3.6));
#8964=CARTESIAN_POINT('',(-2.,-2.44929359829471E-16,3.6));
#8965=CARTESIAN_POINT('',(-2.,-2.44929359829471E-16,3.6));
#8966=CARTESIAN_POINT('Origin',(0.,0.,3.6));
#8967=CARTESIAN_POINT('Origin',(0.,0.,3.6));
#10783=UNCERTAINTY_MEASURE_WITH_UNIT(LENGTH_MEASURE(0.001),#10838,
'DISTANCE_ACCURACY_VALUE',
'Maximum model space distance between geometric entities at asserted c
onnectivities');
#10807=UNCERTAINTY_MEASURE_WITH_UNIT(LENGTH_MEASURE(0.001),#10838,
'DISTANCE_ACCURACY_VALUE',
'Maximum model space distance between geometric entities at asserted c
onnectivities');
#10813=(
GEOMETRIC_REPRESENTATION_CONTEXT(3)
GLOBAL_UNCERTAINTY_ASSIGNED_CONTEXT((#10783))
GLOBAL_UNIT_ASSIGNED_CONTEXT((#10838,#10840,#10841))
REPRESENTATION_CONTEXT('','3D')
);
#10837=(
GEOMETRIC_REPRESENTATION_CONTEXT(3)
GLOBAL_UNCERTAINTY_ASSIGNED_CONTEXT((#10807))
GLOBAL_UNIT_ASSIGNED_CONTEXT((#10838,#10840,#10841))
REPRESENTATION_CONTEXT('','3D')
);
#10838=(
LENGTH_UNIT()
NAMED_UNIT(*)
SI_UNIT(.CENTI.,.METRE.)
);
#10840=(
NAMED_UNIT(*)
PLANE_ANGLE_UNIT()
SI_UNIT($,.RADIAN.)
);
#10841=(
NAMED_UNIT(*)
SI_UNIT($,.STERADIAN.)
SOLID_ANGLE_UNIT()
);
#10847=SHAPE_DEFINITION_REPRESENTATION(#10876,#10946);
#10876=PRODUCT_DEFINITION_SHAPE('',$,#10976);
#10946=SHAPE_REPRESENTATION('',(#6064),#10813);
#10970=PRODUCT_DEFINITION_CONTEXT('part definition',#11059,'design');
#10976=PRODUCT_DEFINITION('Bearing cap','Bearing cap',#11005,#10970);
#11005=PRODUCT_DEFINITION_FORMATION('',$,#11066);
#11059=APPLICATION_CONTEXT(
'Core Data for Automotive Mechanical Design Process');
#11060=PRODUCT_CONTEXT('part definition',#11059,'mechanical');
#11066=PRODUCT('Bearing cap','Bearing cap','Bearing cap',(#11060));
#11160=COLOUR_RGB('Grey',0.48,0.52,0.57);
#11161=FILL_AREA_STYLE_COLOUR('',#11160);
#11162=FILL_AREA_STYLE('',(#11161));
#11163=SURFACE_STYLE_FILL_AREA(#11162);
#11164=SURFACE_SIDE_STYLE('',(#11163));
#11165=SURFACE_STYLE_USAGE(.BOTH.,#11164);
#11166=PRESENTATION_STYLE_ASSIGNMENT((#11165));
ENDSEC;
END-ISO-10303-21;
